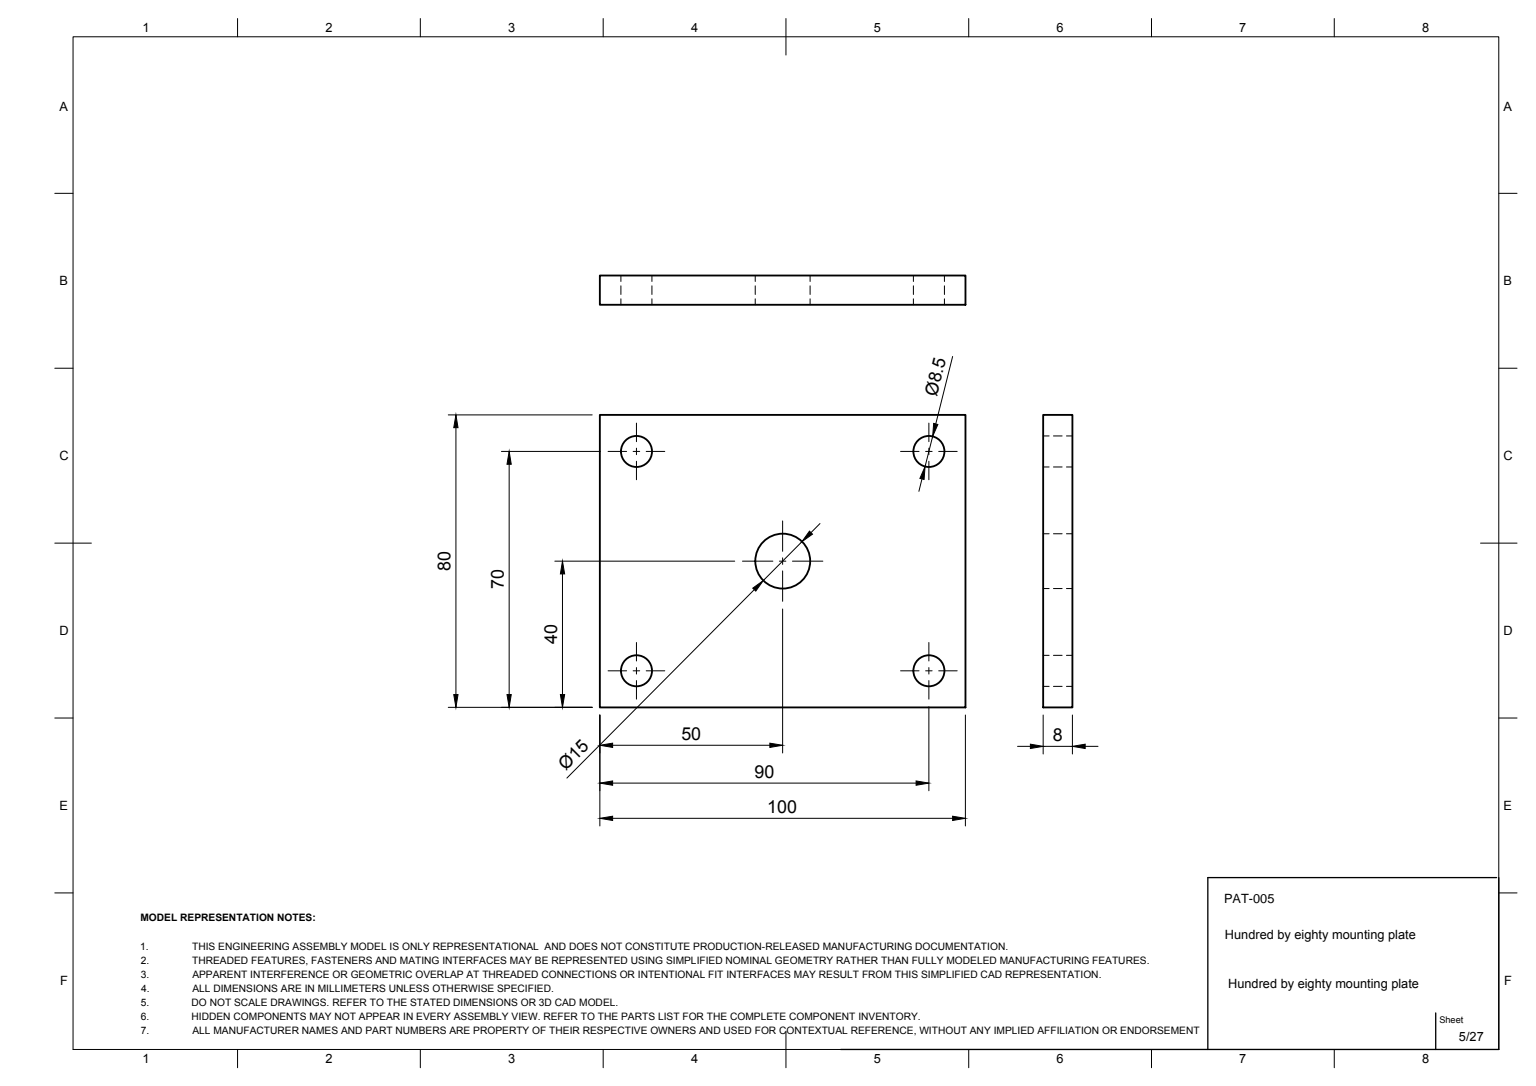
ISO-10303-21;
HEADER;
/* Generated by software containing ST-Developer
 * from STEP Tools, Inc. (www.steptools.com) 
 */

FILE_DESCRIPTION(
/* description */ ('Ball-race swivel caster'),
/* implementation_level */ '2;1');

FILE_NAME(
/* name */ 'Hundred by eighty mounting plate.step',
/* time_stamp */ '2026-10-29T16:15:51-07:00',
/* author */ (''),
/* organization */ (''),
/* preprocessor_version */ 'ST-DEVELOPER v20.2',
/* originating_system */ 'Autodesk Translation Framework v15.17.0.0',
/* authorisation */ '');

FILE_SCHEMA (('AUTOMOTIVE_DESIGN { 1 0 10303 214 3 1 1 }'));
ENDSEC;

DATA;
#10=MECHANICAL_DESIGN_GEOMETRIC_PRESENTATION_REPRESENTATION('',(#298),#7816);
#258=SHAPE_REPRESENTATION_RELATIONSHIP('SRR','None',#7903,#278);
#278=ADVANCED_BREP_SHAPE_REPRESENTATION('',(#334),#7792);
#298=STYLED_ITEM('',(#8111),#334);
#334=MANIFOLD_SOLID_BREP('Body1',#3704);
#369=FACE_BOUND('',#743,.T.);
#370=FACE_BOUND('',#744,.T.);
#371=FACE_BOUND('',#745,.T.);
#372=FACE_BOUND('',#746,.T.);
#373=FACE_BOUND('',#747,.T.);
#374=FACE_BOUND('',#749,.T.);
#375=FACE_BOUND('',#750,.T.);
#376=FACE_BOUND('',#751,.T.);
#377=FACE_BOUND('',#752,.T.);
#378=FACE_BOUND('',#753,.T.);
#438=PLANE('',#3980);
#439=PLANE('',#3981);
#440=PLANE('',#3982);
#441=PLANE('',#3983);
#442=PLANE('',#3984);
#443=PLANE('',#3985);
#524=FACE_OUTER_BOUND('',#733,.T.);
#525=FACE_OUTER_BOUND('',#734,.T.);
#526=FACE_OUTER_BOUND('',#735,.T.);
#527=FACE_OUTER_BOUND('',#736,.T.);
#528=FACE_OUTER_BOUND('',#737,.T.);
#529=FACE_OUTER_BOUND('',#738,.T.);
#530=FACE_OUTER_BOUND('',#739,.T.);
#531=FACE_OUTER_BOUND('',#740,.T.);
#532=FACE_OUTER_BOUND('',#741,.T.);
#533=FACE_OUTER_BOUND('',#742,.T.);
#534=FACE_OUTER_BOUND('',#748,.T.);
#733=EDGE_LOOP('',(#2433,#2434,#2435,#2436));
#734=EDGE_LOOP('',(#2437,#2438,#2439,#2440));
#735=EDGE_LOOP('',(#2441,#2442,#2443,#2444));
#736=EDGE_LOOP('',(#2445,#2446,#2447,#2448));
#737=EDGE_LOOP('',(#2449,#2450,#2451,#2452));
#738=EDGE_LOOP('',(#2453,#2454,#2455,#2456));
#739=EDGE_LOOP('',(#2457,#2458,#2459,#2460));
#740=EDGE_LOOP('',(#2461,#2462,#2463,#2464));
#741=EDGE_LOOP('',(#2465,#2466,#2467,#2468));
#742=EDGE_LOOP('',(#2469,#2470,#2471,#2472));
#743=EDGE_LOOP('',(#2473));
#744=EDGE_LOOP('',(#2474));
#745=EDGE_LOOP('',(#2475));
#746=EDGE_LOOP('',(#2476));
#747=EDGE_LOOP('',(#2477));
#748=EDGE_LOOP('',(#2478,#2479,#2480,#2481));
#749=EDGE_LOOP('',(#2482));
#750=EDGE_LOOP('',(#2483));
#751=EDGE_LOOP('',(#2484));
#752=EDGE_LOOP('',(#2485));
#753=EDGE_LOOP('',(#2486));
#1011=LINE('',#5705,#1166);
#1012=LINE('',#5711,#1167);
#1013=LINE('',#5717,#1168);
#1014=LINE('',#5723,#1169);
#1015=LINE('',#5729,#1170);
#1016=LINE('',#5734,#1171);
#1017=LINE('',#5736,#1172);
#1018=LINE('',#5738,#1173);
#1019=LINE('',#5739,#1174);
#1020=LINE('',#5742,#1175);
#1021=LINE('',#5744,#1176);
#1022=LINE('',#5745,#1177);
#1023=LINE('',#5748,#1178);
#1024=LINE('',#5750,#1179);
#1025=LINE('',#5751,#1180);
#1026=LINE('',#5753,#1181);
#1027=LINE('',#5754,#1182);
#1166=VECTOR('',#4499,0.75);
#1167=VECTOR('',#4506,0.425);
#1168=VECTOR('',#4513,0.425);
#1169=VECTOR('',#4520,0.425);
#1170=VECTOR('',#4527,0.425);
#1171=VECTOR('',#4532,1.);
#1172=VECTOR('',#4533,1.);
#1173=VECTOR('',#4534,1.);
#1174=VECTOR('',#4535,1.);
#1175=VECTOR('',#4538,1.);
#1176=VECTOR('',#4539,1.);
#1177=VECTOR('',#4540,1.);
#1178=VECTOR('',#4543,1.);
#1179=VECTOR('',#4544,1.);
#1180=VECTOR('',#4545,1.);
#1181=VECTOR('',#4548,1.);
#1182=VECTOR('',#4549,1.);
#1321=CIRCLE('',#3966,0.75);
#1322=CIRCLE('',#3967,0.75);
#1323=CIRCLE('',#3969,0.425);
#1324=CIRCLE('',#3970,0.425);
#1325=CIRCLE('',#3972,0.425);
#1326=CIRCLE('',#3973,0.425);
#1327=CIRCLE('',#3975,0.425);
#1328=CIRCLE('',#3976,0.425);
#1329=CIRCLE('',#3978,0.425);
#1330=CIRCLE('',#3979,0.425);
#1585=VERTEX_POINT('',#5702);
#1586=VERTEX_POINT('',#5704);
#1587=VERTEX_POINT('',#5708);
#1588=VERTEX_POINT('',#5710);
#1589=VERTEX_POINT('',#5714);
#1590=VERTEX_POINT('',#5716);
#1591=VERTEX_POINT('',#5720);
#1592=VERTEX_POINT('',#5722);
#1593=VERTEX_POINT('',#5726);
#1594=VERTEX_POINT('',#5728);
#1595=VERTEX_POINT('',#5732);
#1596=VERTEX_POINT('',#5733);
#1597=VERTEX_POINT('',#5735);
#1598=VERTEX_POINT('',#5737);
#1599=VERTEX_POINT('',#5741);
#1600=VERTEX_POINT('',#5743);
#1601=VERTEX_POINT('',#5747);
#1602=VERTEX_POINT('',#5749);
#1936=EDGE_CURVE('',#1585,#1585,#1321,.T.);
#1937=EDGE_CURVE('',#1585,#1586,#1011,.T.);
#1938=EDGE_CURVE('',#1586,#1586,#1322,.T.);
#1939=EDGE_CURVE('',#1587,#1587,#1323,.T.);
#1940=EDGE_CURVE('',#1587,#1588,#1012,.T.);
#1941=EDGE_CURVE('',#1588,#1588,#1324,.T.);
#1942=EDGE_CURVE('',#1589,#1589,#1325,.T.);
#1943=EDGE_CURVE('',#1589,#1590,#1013,.T.);
#1944=EDGE_CURVE('',#1590,#1590,#1326,.T.);
#1945=EDGE_CURVE('',#1591,#1591,#1327,.T.);
#1946=EDGE_CURVE('',#1591,#1592,#1014,.T.);
#1947=EDGE_CURVE('',#1592,#1592,#1328,.T.);
#1948=EDGE_CURVE('',#1593,#1593,#1329,.T.);
#1949=EDGE_CURVE('',#1593,#1594,#1015,.T.);
#1950=EDGE_CURVE('',#1594,#1594,#1330,.T.);
#1951=EDGE_CURVE('',#1595,#1596,#1016,.T.);
#1952=EDGE_CURVE('',#1596,#1597,#1017,.T.);
#1953=EDGE_CURVE('',#1598,#1597,#1018,.T.);
#1954=EDGE_CURVE('',#1595,#1598,#1019,.T.);
#1955=EDGE_CURVE('',#1599,#1595,#1020,.T.);
#1956=EDGE_CURVE('',#1600,#1598,#1021,.T.);
#1957=EDGE_CURVE('',#1599,#1600,#1022,.T.);
#1958=EDGE_CURVE('',#1601,#1599,#1023,.T.);
#1959=EDGE_CURVE('',#1602,#1600,#1024,.T.);
#1960=EDGE_CURVE('',#1601,#1602,#1025,.T.);
#1961=EDGE_CURVE('',#1596,#1601,#1026,.T.);
#1962=EDGE_CURVE('',#1597,#1602,#1027,.T.);
#2433=ORIENTED_EDGE('',*,*,#1936,.F.);
#2434=ORIENTED_EDGE('',*,*,#1937,.T.);
#2435=ORIENTED_EDGE('',*,*,#1938,.F.);
#2436=ORIENTED_EDGE('',*,*,#1937,.F.);
#2437=ORIENTED_EDGE('',*,*,#1939,.F.);
#2438=ORIENTED_EDGE('',*,*,#1940,.T.);
#2439=ORIENTED_EDGE('',*,*,#1941,.F.);
#2440=ORIENTED_EDGE('',*,*,#1940,.F.);
#2441=ORIENTED_EDGE('',*,*,#1942,.F.);
#2442=ORIENTED_EDGE('',*,*,#1943,.T.);
#2443=ORIENTED_EDGE('',*,*,#1944,.F.);
#2444=ORIENTED_EDGE('',*,*,#1943,.F.);
#2445=ORIENTED_EDGE('',*,*,#1945,.F.);
#2446=ORIENTED_EDGE('',*,*,#1946,.T.);
#2447=ORIENTED_EDGE('',*,*,#1947,.F.);
#2448=ORIENTED_EDGE('',*,*,#1946,.F.);
#2449=ORIENTED_EDGE('',*,*,#1948,.F.);
#2450=ORIENTED_EDGE('',*,*,#1949,.T.);
#2451=ORIENTED_EDGE('',*,*,#1950,.F.);
#2452=ORIENTED_EDGE('',*,*,#1949,.F.);
#2453=ORIENTED_EDGE('',*,*,#1951,.T.);
#2454=ORIENTED_EDGE('',*,*,#1952,.T.);
#2455=ORIENTED_EDGE('',*,*,#1953,.F.);
#2456=ORIENTED_EDGE('',*,*,#1954,.F.);
#2457=ORIENTED_EDGE('',*,*,#1955,.T.);
#2458=ORIENTED_EDGE('',*,*,#1954,.T.);
#2459=ORIENTED_EDGE('',*,*,#1956,.F.);
#2460=ORIENTED_EDGE('',*,*,#1957,.F.);
#2461=ORIENTED_EDGE('',*,*,#1958,.T.);
#2462=ORIENTED_EDGE('',*,*,#1957,.T.);
#2463=ORIENTED_EDGE('',*,*,#1959,.F.);
#2464=ORIENTED_EDGE('',*,*,#1960,.F.);
#2465=ORIENTED_EDGE('',*,*,#1961,.T.);
#2466=ORIENTED_EDGE('',*,*,#1960,.T.);
#2467=ORIENTED_EDGE('',*,*,#1962,.F.);
#2468=ORIENTED_EDGE('',*,*,#1952,.F.);
#2469=ORIENTED_EDGE('',*,*,#1962,.T.);
#2470=ORIENTED_EDGE('',*,*,#1959,.T.);
#2471=ORIENTED_EDGE('',*,*,#1956,.T.);
#2472=ORIENTED_EDGE('',*,*,#1953,.T.);
#2473=ORIENTED_EDGE('',*,*,#1938,.T.);
#2474=ORIENTED_EDGE('',*,*,#1941,.T.);
#2475=ORIENTED_EDGE('',*,*,#1944,.T.);
#2476=ORIENTED_EDGE('',*,*,#1947,.T.);
#2477=ORIENTED_EDGE('',*,*,#1950,.T.);
#2478=ORIENTED_EDGE('',*,*,#1961,.F.);
#2479=ORIENTED_EDGE('',*,*,#1951,.F.);
#2480=ORIENTED_EDGE('',*,*,#1955,.F.);
#2481=ORIENTED_EDGE('',*,*,#1958,.F.);
#2482=ORIENTED_EDGE('',*,*,#1936,.T.);
#2483=ORIENTED_EDGE('',*,*,#1939,.T.);
#2484=ORIENTED_EDGE('',*,*,#1942,.T.);
#2485=ORIENTED_EDGE('',*,*,#1945,.T.);
#2486=ORIENTED_EDGE('',*,*,#1948,.T.);
#3427=CYLINDRICAL_SURFACE('',#3965,0.75);
#3428=CYLINDRICAL_SURFACE('',#3968,0.425);
#3429=CYLINDRICAL_SURFACE('',#3971,0.425);
#3430=CYLINDRICAL_SURFACE('',#3974,0.425);
#3431=CYLINDRICAL_SURFACE('',#3977,0.425);
#3495=ADVANCED_FACE('',(#524),#3427,.F.);
#3496=ADVANCED_FACE('',(#525),#3428,.F.);
#3497=ADVANCED_FACE('',(#526),#3429,.F.);
#3498=ADVANCED_FACE('',(#527),#3430,.F.);
#3499=ADVANCED_FACE('',(#528),#3431,.F.);
#3500=ADVANCED_FACE('',(#529),#438,.T.);
#3501=ADVANCED_FACE('',(#530),#439,.T.);
#3502=ADVANCED_FACE('',(#531),#440,.T.);
#3503=ADVANCED_FACE('',(#532),#441,.T.);
#3504=ADVANCED_FACE('',(#533,#369,#370,#371,#372,#373),#442,.T.);
#3505=ADVANCED_FACE('',(#534,#374,#375,#376,#377,#378),#443,.F.);
#3704=CLOSED_SHELL('',(#3495,#3496,#3497,#3498,#3499,#3500,#3501,#3502,
#3503,#3504,#3505));
#3964=AXIS2_PLACEMENT_3D('',#5700,#4493,#4494);
#3965=AXIS2_PLACEMENT_3D('',#5701,#4495,#4496);
#3966=AXIS2_PLACEMENT_3D('',#5703,#4497,#4498);
#3967=AXIS2_PLACEMENT_3D('',#5706,#4500,#4501);
#3968=AXIS2_PLACEMENT_3D('',#5707,#4502,#4503);
#3969=AXIS2_PLACEMENT_3D('',#5709,#4504,#4505);
#3970=AXIS2_PLACEMENT_3D('',#5712,#4507,#4508);
#3971=AXIS2_PLACEMENT_3D('',#5713,#4509,#4510);
#3972=AXIS2_PLACEMENT_3D('',#5715,#4511,#4512);
#3973=AXIS2_PLACEMENT_3D('',#5718,#4514,#4515);
#3974=AXIS2_PLACEMENT_3D('',#5719,#4516,#4517);
#3975=AXIS2_PLACEMENT_3D('',#5721,#4518,#4519);
#3976=AXIS2_PLACEMENT_3D('',#5724,#4521,#4522);
#3977=AXIS2_PLACEMENT_3D('',#5725,#4523,#4524);
#3978=AXIS2_PLACEMENT_3D('',#5727,#4525,#4526);
#3979=AXIS2_PLACEMENT_3D('',#5730,#4528,#4529);
#3980=AXIS2_PLACEMENT_3D('',#5731,#4530,#4531);
#3981=AXIS2_PLACEMENT_3D('',#5740,#4536,#4537);
#3982=AXIS2_PLACEMENT_3D('',#5746,#4541,#4542);
#3983=AXIS2_PLACEMENT_3D('',#5752,#4546,#4547);
#3984=AXIS2_PLACEMENT_3D('',#5755,#4550,#4551);
#3985=AXIS2_PLACEMENT_3D('',#5756,#4552,#4553);
#4493=DIRECTION('axis',(0.,0.,1.));
#4494=DIRECTION('refdir',(1.,0.,0.));
#4495=DIRECTION('center_axis',(0.,0.,1.));
#4496=DIRECTION('ref_axis',(1.,0.,0.));
#4497=DIRECTION('center_axis',(0.,0.,1.));
#4498=DIRECTION('ref_axis',(1.,0.,0.));
#4499=DIRECTION('',(0.,0.,1.));
#4500=DIRECTION('center_axis',(0.,0.,-1.));
#4501=DIRECTION('ref_axis',(1.,0.,0.));
#4502=DIRECTION('center_axis',(0.,0.,1.));
#4503=DIRECTION('ref_axis',(1.,0.,0.));
#4504=DIRECTION('center_axis',(0.,0.,1.));
#4505=DIRECTION('ref_axis',(1.,0.,0.));
#4506=DIRECTION('',(0.,0.,1.));
#4507=DIRECTION('center_axis',(0.,0.,-1.));
#4508=DIRECTION('ref_axis',(1.,0.,0.));
#4509=DIRECTION('center_axis',(0.,0.,1.));
#4510=DIRECTION('ref_axis',(1.,0.,0.));
#4511=DIRECTION('center_axis',(0.,0.,1.));
#4512=DIRECTION('ref_axis',(1.,0.,0.));
#4513=DIRECTION('',(0.,0.,1.));
#4514=DIRECTION('center_axis',(0.,0.,-1.));
#4515=DIRECTION('ref_axis',(1.,0.,0.));
#4516=DIRECTION('center_axis',(0.,0.,1.));
#4517=DIRECTION('ref_axis',(1.,0.,0.));
#4518=DIRECTION('center_axis',(0.,0.,1.));
#4519=DIRECTION('ref_axis',(1.,0.,0.));
#4520=DIRECTION('',(0.,0.,1.));
#4521=DIRECTION('center_axis',(0.,0.,-1.));
#4522=DIRECTION('ref_axis',(1.,0.,0.));
#4523=DIRECTION('center_axis',(0.,0.,1.));
#4524=DIRECTION('ref_axis',(1.,0.,0.));
#4525=DIRECTION('center_axis',(0.,0.,1.));
#4526=DIRECTION('ref_axis',(1.,0.,0.));
#4527=DIRECTION('',(0.,0.,1.));
#4528=DIRECTION('center_axis',(0.,0.,-1.));
#4529=DIRECTION('ref_axis',(1.,0.,0.));
#4530=DIRECTION('center_axis',(0.,1.,0.));
#4531=DIRECTION('ref_axis',(-1.,0.,0.));
#4532=DIRECTION('',(-1.,0.,0.));
#4533=DIRECTION('',(0.,0.,1.));
#4534=DIRECTION('',(-1.,0.,0.));
#4535=DIRECTION('',(0.,0.,1.));
#4536=DIRECTION('center_axis',(1.,0.,0.));
#4537=DIRECTION('ref_axis',(0.,1.,0.));
#4538=DIRECTION('',(0.,1.,0.));
#4539=DIRECTION('',(0.,1.,0.));
#4540=DIRECTION('',(0.,0.,1.));
#4541=DIRECTION('center_axis',(0.,-1.,0.));
#4542=DIRECTION('ref_axis',(1.,0.,0.));
#4543=DIRECTION('',(1.,0.,0.));
#4544=DIRECTION('',(1.,0.,0.));
#4545=DIRECTION('',(0.,0.,1.));
#4546=DIRECTION('center_axis',(-1.,0.,0.));
#4547=DIRECTION('ref_axis',(0.,-1.,0.));
#4548=DIRECTION('',(0.,-1.,0.));
#4549=DIRECTION('',(0.,-1.,0.));
#4550=DIRECTION('center_axis',(0.,0.,1.));
#4551=DIRECTION('ref_axis',(1.,0.,0.));
#4552=DIRECTION('center_axis',(0.,0.,1.));
#4553=DIRECTION('ref_axis',(1.,0.,0.));
#5700=CARTESIAN_POINT('',(0.,0.,0.));
#5701=CARTESIAN_POINT('Origin',(-2.,0.,10.1));
#5702=CARTESIAN_POINT('',(-2.75,-9.18485099360515E-17,10.2));
#5703=CARTESIAN_POINT('Origin',(-2.,0.,10.2));
#5704=CARTESIAN_POINT('',(-2.75,9.18485099360515E-17,11.));
#5705=CARTESIAN_POINT('',(-2.75,-9.18485099360515E-17,10.1));
#5706=CARTESIAN_POINT('Origin',(-2.,0.,11.));
#5707=CARTESIAN_POINT('Origin',(2.,-3.,10.1));
#5708=CARTESIAN_POINT('',(1.575,-3.,10.2));
#5709=CARTESIAN_POINT('Origin',(2.,-3.,10.2));
#5710=CARTESIAN_POINT('',(1.575,-3.,11.));
#5711=CARTESIAN_POINT('',(1.575,-3.,10.1));
#5712=CARTESIAN_POINT('Origin',(2.,-3.,11.));
#5713=CARTESIAN_POINT('Origin',(-6.,3.,10.1));
#5714=CARTESIAN_POINT('',(-6.425,3.,10.2));
#5715=CARTESIAN_POINT('Origin',(-6.,3.,10.2));
#5716=CARTESIAN_POINT('',(-6.425,3.,11.));
#5717=CARTESIAN_POINT('',(-6.425,3.,10.1));
#5718=CARTESIAN_POINT('Origin',(-6.,3.,11.));
#5719=CARTESIAN_POINT('Origin',(-6.,-3.,10.1));
#5720=CARTESIAN_POINT('',(-6.425,-3.,10.2));
#5721=CARTESIAN_POINT('Origin',(-6.,-3.,10.2));
#5722=CARTESIAN_POINT('',(-6.425,-3.,11.));
#5723=CARTESIAN_POINT('',(-6.425,-3.,10.1));
#5724=CARTESIAN_POINT('Origin',(-6.,-3.,11.));
#5725=CARTESIAN_POINT('Origin',(2.,3.,10.1));
#5726=CARTESIAN_POINT('',(1.575,3.,10.2));
#5727=CARTESIAN_POINT('Origin',(2.,3.,10.2));
#5728=CARTESIAN_POINT('',(1.575,3.,11.));
#5729=CARTESIAN_POINT('',(1.575,3.,10.1));
#5730=CARTESIAN_POINT('Origin',(2.,3.,11.));
#5731=CARTESIAN_POINT('Origin',(3.,4.,10.2));
#5732=CARTESIAN_POINT('',(3.,4.,10.2));
#5733=CARTESIAN_POINT('',(-7.,4.,10.2));
#5734=CARTESIAN_POINT('',(3.,4.,10.2));
#5735=CARTESIAN_POINT('',(-7.,4.,11.));
#5736=CARTESIAN_POINT('',(-7.,4.,10.2));
#5737=CARTESIAN_POINT('',(3.,4.,11.));
#5738=CARTESIAN_POINT('',(3.,4.,11.));
#5739=CARTESIAN_POINT('',(3.,4.,10.2));
#5740=CARTESIAN_POINT('Origin',(3.,-4.,10.2));
#5741=CARTESIAN_POINT('',(3.,-4.,10.2));
#5742=CARTESIAN_POINT('',(3.,-4.,10.2));
#5743=CARTESIAN_POINT('',(3.,-4.,11.));
#5744=CARTESIAN_POINT('',(3.,-4.,11.));
#5745=CARTESIAN_POINT('',(3.,-4.,10.2));
#5746=CARTESIAN_POINT('Origin',(-7.,-4.,10.2));
#5747=CARTESIAN_POINT('',(-7.,-4.,10.2));
#5748=CARTESIAN_POINT('',(-7.,-4.,10.2));
#5749=CARTESIAN_POINT('',(-7.,-4.,11.));
#5750=CARTESIAN_POINT('',(-7.,-4.,11.));
#5751=CARTESIAN_POINT('',(-7.,-4.,10.2));
#5752=CARTESIAN_POINT('Origin',(-7.,4.,10.2));
#5753=CARTESIAN_POINT('',(-7.,4.,10.2));
#5754=CARTESIAN_POINT('',(-7.,4.,11.));
#5755=CARTESIAN_POINT('Origin',(-2.,0.,11.));
#5756=CARTESIAN_POINT('Origin',(-2.,0.,10.2));
#7765=UNCERTAINTY_MEASURE_WITH_UNIT(LENGTH_MEASURE(0.001),#7817,
'DISTANCE_ACCURACY_VALUE',
'Maximum model space distance between geometric entities at asserted c
onnectivities');
#7789=UNCERTAINTY_MEASURE_WITH_UNIT(LENGTH_MEASURE(0.001),#7817,
'DISTANCE_ACCURACY_VALUE',
'Maximum model space distance between geometric entities at asserted c
onnectivities');
#7792=(
GEOMETRIC_REPRESENTATION_CONTEXT(3)
GLOBAL_UNCERTAINTY_ASSIGNED_CONTEXT((#7765))
GLOBAL_UNIT_ASSIGNED_CONTEXT((#7817,#7819,#7820))
REPRESENTATION_CONTEXT('','3D')
);
#7816=(
GEOMETRIC_REPRESENTATION_CONTEXT(3)
GLOBAL_UNCERTAINTY_ASSIGNED_CONTEXT((#7789))
GLOBAL_UNIT_ASSIGNED_CONTEXT((#7817,#7819,#7820))
REPRESENTATION_CONTEXT('','3D')
);
#7817=(
LENGTH_UNIT()
NAMED_UNIT(*)
SI_UNIT(.CENTI.,.METRE.)
);
#7819=(
NAMED_UNIT(*)
PLANE_ANGLE_UNIT()
SI_UNIT($,.RADIAN.)
);
#7820=(
NAMED_UNIT(*)
SI_UNIT($,.STERADIAN.)
SOLID_ANGLE_UNIT()
);
#7823=SHAPE_DEFINITION_REPRESENTATION(#7849,#7903);
#7849=PRODUCT_DEFINITION_SHAPE('',$,#7930);
#7903=SHAPE_REPRESENTATION('',(#3964),#7792);
#7927=PRODUCT_DEFINITION_CONTEXT('part definition',#8007,'design');
#7930=PRODUCT_DEFINITION('Hundred by eighty mounting plate',
'Hundred by eighty mounting plate',#7956,#7927);
#7956=PRODUCT_DEFINITION_FORMATION('',$,#8011);
#8007=APPLICATION_CONTEXT(
'Core Data for Automotive Mechanical Design Process');
#8008=PRODUCT_CONTEXT('part definition',#8007,'mechanical');
#8011=PRODUCT('Hundred by eighty mounting plate',
'Hundred by eighty mounting plate','Hundred by eighty mounting plate',(#8008));
#8105=COLOUR_RGB('Off White',0.89,0.88,0.83);
#8106=FILL_AREA_STYLE_COLOUR('',#8105);
#8107=FILL_AREA_STYLE('',(#8106));
#8108=SURFACE_STYLE_FILL_AREA(#8107);
#8109=SURFACE_SIDE_STYLE('',(#8108));
#8110=SURFACE_STYLE_USAGE(.BOTH.,#8109);
#8111=PRESENTATION_STYLE_ASSIGNMENT((#8110));
ENDSEC;
END-ISO-10303-21;
